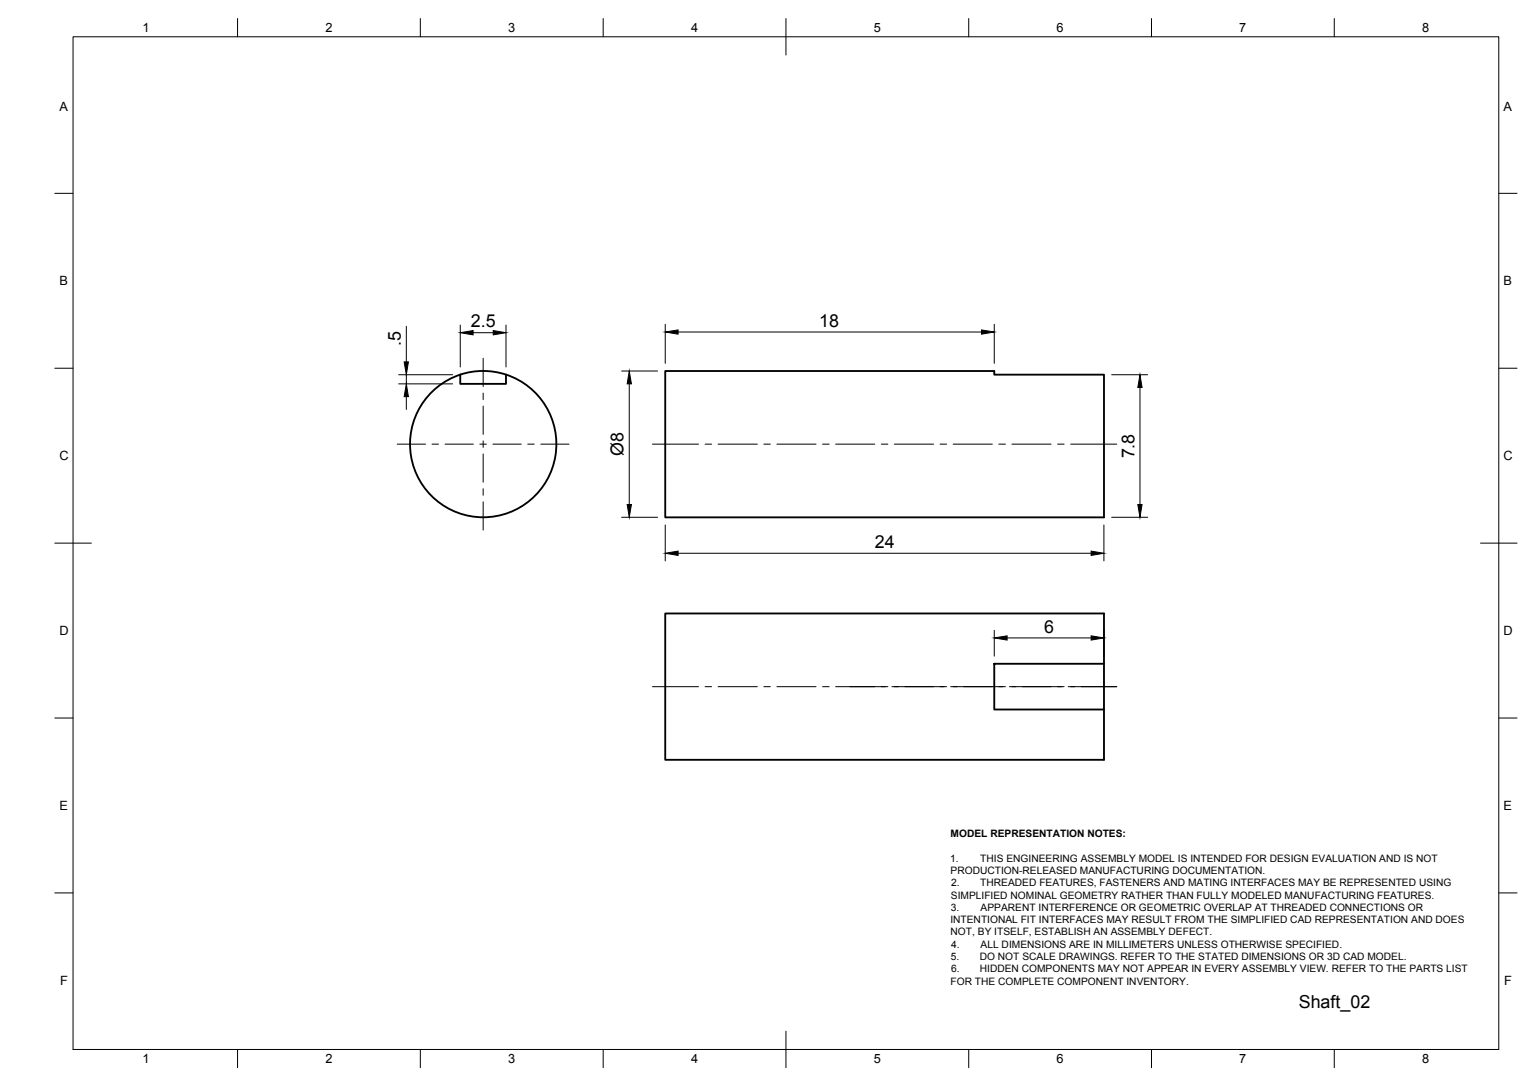
ISO-10303-21;
HEADER;
/* Generated by software containing ST-Developer
 * from STEP Tools, Inc. (www.steptools.com) 
 */

FILE_DESCRIPTION(
/* description */ (''),
/* implementation_level */ '2;1');

FILE_NAME(
/* name */ 'Shaft_02.step',
/* time_stamp */ '2026-10-05T22:24:12-07:00',
/* author */ (''),
/* organization */ (''),
/* preprocessor_version */ 'ST-DEVELOPER v20.2',
/* originating_system */ 'Autodesk Translation Framework v15.15.0.0',
/* authorisation */ '');

FILE_SCHEMA (('AUTOMOTIVE_DESIGN { 1 0 10303 214 3 1 1 }'));
ENDSEC;

DATA;
#10=MECHANICAL_DESIGN_GEOMETRIC_PRESENTATION_REPRESENTATION('',(#56),#2116);
#42=SHAPE_REPRESENTATION_RELATIONSHIP('SRR','None',#2148,#49);
#49=ADVANCED_BREP_SHAPE_REPRESENTATION('',(#63),#2112);
#56=STYLED_ITEM('',(#2192),#63);
#63=MANIFOLD_SOLID_BREP('Body1',#1150);
#107=PLANE('',#1310);
#108=PLANE('',#1311);
#109=PLANE('',#1312);
#110=PLANE('',#1313);
#111=PLANE('',#1315);
#112=PLANE('',#1320);
#172=FACE_OUTER_BOUND('',#247,.T.);
#173=FACE_OUTER_BOUND('',#248,.T.);
#174=FACE_OUTER_BOUND('',#249,.T.);
#175=FACE_OUTER_BOUND('',#250,.T.);
#176=FACE_OUTER_BOUND('',#251,.T.);
#177=FACE_OUTER_BOUND('',#252,.T.);
#178=FACE_OUTER_BOUND('',#253,.T.);
#247=EDGE_LOOP('',(#961,#962,#963,#964));
#248=EDGE_LOOP('',(#965,#966,#967,#968));
#249=EDGE_LOOP('',(#969,#970,#971,#972));
#250=EDGE_LOOP('',(#973,#974,#975,#976));
#251=EDGE_LOOP('',(#977,#978,#979,#980,#981));
#252=EDGE_LOOP('',(#982,#983,#984,#985,#986,#987,#988,#989));
#253=EDGE_LOOP('',(#990));
#335=LINE('',#1976,#440);
#336=LINE('',#1978,#441);
#337=LINE('',#1980,#442);
#338=LINE('',#1981,#443);
#339=LINE('',#1984,#444);
#340=LINE('',#1986,#445);
#341=LINE('',#1987,#446);
#342=LINE('',#1991,#447);
#343=LINE('',#1992,#448);
#344=LINE('',#1993,#449);
#345=LINE('',#2002,#450);
#440=VECTOR('',#1571,10.);
#441=VECTOR('',#1572,10.);
#442=VECTOR('',#1573,10.);
#443=VECTOR('',#1574,10.);
#444=VECTOR('',#1577,10.);
#445=VECTOR('',#1578,10.);
#446=VECTOR('',#1579,10.);
#447=VECTOR('',#1582,10.);
#448=VECTOR('',#1583,10.);
#449=VECTOR('',#1584,10.);
#450=VECTOR('',#1597,4.);
#518=CIRCLE('',#1314,4.);
#519=CIRCLE('',#1316,4.);
#520=CIRCLE('',#1317,4.);
#521=CIRCLE('',#1319,4.);
#589=VERTEX_POINT('',#1974);
#590=VERTEX_POINT('',#1975);
#591=VERTEX_POINT('',#1977);
#592=VERTEX_POINT('',#1979);
#593=VERTEX_POINT('',#1983);
#594=VERTEX_POINT('',#1985);
#595=VERTEX_POINT('',#1989);
#596=VERTEX_POINT('',#1990);
#597=VERTEX_POINT('',#1997);
#598=VERTEX_POINT('',#2001);
#719=EDGE_CURVE('',#589,#590,#335,.T.);
#720=EDGE_CURVE('',#591,#589,#336,.T.);
#721=EDGE_CURVE('',#592,#591,#337,.T.);
#722=EDGE_CURVE('',#590,#592,#338,.T.);
#723=EDGE_CURVE('',#592,#593,#339,.T.);
#724=EDGE_CURVE('',#594,#591,#340,.T.);
#725=EDGE_CURVE('',#593,#594,#341,.T.);
#726=EDGE_CURVE('',#595,#596,#342,.T.);
#727=EDGE_CURVE('',#593,#595,#343,.T.);
#728=EDGE_CURVE('',#596,#594,#344,.T.);
#729=EDGE_CURVE('',#596,#589,#518,.T.);
#730=EDGE_CURVE('',#595,#597,#519,.T.);
#731=EDGE_CURVE('',#597,#590,#520,.T.);
#732=EDGE_CURVE('',#597,#598,#345,.T.);
#733=EDGE_CURVE('',#598,#598,#521,.T.);
#961=ORIENTED_EDGE('',*,*,#719,.F.);
#962=ORIENTED_EDGE('',*,*,#720,.F.);
#963=ORIENTED_EDGE('',*,*,#721,.F.);
#964=ORIENTED_EDGE('',*,*,#722,.F.);
#965=ORIENTED_EDGE('',*,*,#723,.F.);
#966=ORIENTED_EDGE('',*,*,#721,.T.);
#967=ORIENTED_EDGE('',*,*,#724,.F.);
#968=ORIENTED_EDGE('',*,*,#725,.F.);
#969=ORIENTED_EDGE('',*,*,#726,.F.);
#970=ORIENTED_EDGE('',*,*,#727,.F.);
#971=ORIENTED_EDGE('',*,*,#725,.T.);
#972=ORIENTED_EDGE('',*,*,#728,.F.);
#973=ORIENTED_EDGE('',*,*,#729,.F.);
#974=ORIENTED_EDGE('',*,*,#728,.T.);
#975=ORIENTED_EDGE('',*,*,#724,.T.);
#976=ORIENTED_EDGE('',*,*,#720,.T.);
#977=ORIENTED_EDGE('',*,*,#722,.T.);
#978=ORIENTED_EDGE('',*,*,#723,.T.);
#979=ORIENTED_EDGE('',*,*,#727,.T.);
#980=ORIENTED_EDGE('',*,*,#730,.T.);
#981=ORIENTED_EDGE('',*,*,#731,.T.);
#982=ORIENTED_EDGE('',*,*,#730,.F.);
#983=ORIENTED_EDGE('',*,*,#726,.T.);
#984=ORIENTED_EDGE('',*,*,#729,.T.);
#985=ORIENTED_EDGE('',*,*,#719,.T.);
#986=ORIENTED_EDGE('',*,*,#731,.F.);
#987=ORIENTED_EDGE('',*,*,#732,.T.);
#988=ORIENTED_EDGE('',*,*,#733,.T.);
#989=ORIENTED_EDGE('',*,*,#732,.F.);
#990=ORIENTED_EDGE('',*,*,#733,.F.);
#1078=CYLINDRICAL_SURFACE('',#1318,4.);
#1121=ADVANCED_FACE('',(#172),#107,.T.);
#1122=ADVANCED_FACE('',(#173),#108,.T.);
#1123=ADVANCED_FACE('',(#174),#109,.T.);
#1124=ADVANCED_FACE('',(#175),#110,.T.);
#1125=ADVANCED_FACE('',(#176),#111,.T.);
#1126=ADVANCED_FACE('',(#177),#1078,.T.);
#1127=ADVANCED_FACE('',(#178),#112,.F.);
#1150=CLOSED_SHELL('',(#1121,#1122,#1123,#1124,#1125,#1126,#1127));
#1309=AXIS2_PLACEMENT_3D('',#1972,#1567,#1568);
#1310=AXIS2_PLACEMENT_3D('',#1973,#1569,#1570);
#1311=AXIS2_PLACEMENT_3D('',#1982,#1575,#1576);
#1312=AXIS2_PLACEMENT_3D('',#1988,#1580,#1581);
#1313=AXIS2_PLACEMENT_3D('',#1994,#1585,#1586);
#1314=AXIS2_PLACEMENT_3D('',#1995,#1587,#1588);
#1315=AXIS2_PLACEMENT_3D('',#1996,#1589,#1590);
#1316=AXIS2_PLACEMENT_3D('',#1998,#1591,#1592);
#1317=AXIS2_PLACEMENT_3D('',#1999,#1593,#1594);
#1318=AXIS2_PLACEMENT_3D('',#2000,#1595,#1596);
#1319=AXIS2_PLACEMENT_3D('',#2003,#1598,#1599);
#1320=AXIS2_PLACEMENT_3D('',#2004,#1600,#1601);
#1567=DIRECTION('axis',(0.,0.,1.));
#1568=DIRECTION('refdir',(1.,0.,0.));
#1569=DIRECTION('center_axis',(-1.,0.,0.));
#1570=DIRECTION('ref_axis',(0.,0.,1.));
#1571=DIRECTION('',(0.,-1.,0.));
#1572=DIRECTION('',(0.,0.,1.));
#1573=DIRECTION('',(0.,1.,0.));
#1574=DIRECTION('',(0.,0.,-1.));
#1575=DIRECTION('center_axis',(0.,0.,1.));
#1576=DIRECTION('ref_axis',(1.,0.,0.));
#1577=DIRECTION('',(-1.,0.,0.));
#1578=DIRECTION('',(1.,0.,0.));
#1579=DIRECTION('',(0.,1.,0.));
#1580=DIRECTION('center_axis',(1.,0.,0.));
#1581=DIRECTION('ref_axis',(0.,0.,-1.));
#1582=DIRECTION('',(0.,1.,0.));
#1583=DIRECTION('',(0.,0.,1.));
#1584=DIRECTION('',(0.,0.,-1.));
#1585=DIRECTION('center_axis',(0.,-1.,0.));
#1586=DIRECTION('ref_axis',(0.,0.,-1.));
#1587=DIRECTION('center_axis',(0.,1.,0.));
#1588=DIRECTION('ref_axis',(1.,0.,0.));
#1589=DIRECTION('center_axis',(0.,-1.,0.));
#1590=DIRECTION('ref_axis',(1.,0.,0.));
#1591=DIRECTION('center_axis',(0.,-1.,0.));
#1592=DIRECTION('ref_axis',(1.,0.,0.));
#1593=DIRECTION('center_axis',(0.,-1.,0.));
#1594=DIRECTION('ref_axis',(1.,0.,0.));
#1595=DIRECTION('center_axis',(0.,-1.,0.));
#1596=DIRECTION('ref_axis',(1.,0.,0.));
#1597=DIRECTION('',(0.,1.,0.));
#1598=DIRECTION('center_axis',(0.,-1.,0.));
#1599=DIRECTION('ref_axis',(1.,0.,0.));
#1600=DIRECTION('center_axis',(0.,-1.,0.));
#1601=DIRECTION('ref_axis',(1.,0.,0.));
#1972=CARTESIAN_POINT('',(0.,0.,0.));
#1973=CARTESIAN_POINT('Origin',(3.25,10.,5.29967103839267));
#1974=CARTESIAN_POINT('',(3.25,16.,5.79967103839267));
#1975=CARTESIAN_POINT('',(3.25,10.,5.79967103839267));
#1976=CARTESIAN_POINT('',(3.25,10.,5.79967103839267));
#1977=CARTESIAN_POINT('',(3.25,16.,5.29967103839267));
#1978=CARTESIAN_POINT('',(3.25,16.,8.32461990770089));
#1979=CARTESIAN_POINT('',(3.25,10.,5.29967103839267));
#1980=CARTESIAN_POINT('',(3.25,10.,5.29967103839267));
#1981=CARTESIAN_POINT('',(3.25,10.,3.64983551919633));
#1982=CARTESIAN_POINT('Origin',(0.75,10.,5.29967103839267));
#1983=CARTESIAN_POINT('',(0.75,10.,5.29967103839267));
#1984=CARTESIAN_POINT('',(1.375,10.,5.29967103839267));
#1985=CARTESIAN_POINT('',(0.75,16.,5.29967103839267));
#1986=CARTESIAN_POINT('',(0.75,16.,5.29967103839267));
#1987=CARTESIAN_POINT('',(0.75,10.,5.29967103839267));
#1988=CARTESIAN_POINT('Origin',(0.75,10.,6.84122918275927));
#1989=CARTESIAN_POINT('',(0.75,10.,5.79967103839267));
#1990=CARTESIAN_POINT('',(0.75,16.,5.79967103839267));
#1991=CARTESIAN_POINT('',(0.75,10.,5.79967103839267));
#1992=CARTESIAN_POINT('',(0.75,10.,4.42061459137964));
#1993=CARTESIAN_POINT('',(0.75,16.,5.79967103839267));
#1994=CARTESIAN_POINT('Origin',(2.,16.,6.07045011057597));
#1995=CARTESIAN_POINT('Origin',(2.,16.,2.));
#1996=CARTESIAN_POINT('Origin',(2.,10.,2.));
#1997=CARTESIAN_POINT('',(-2.,10.,2.));
#1998=CARTESIAN_POINT('Origin',(2.,10.,2.));
#1999=CARTESIAN_POINT('Origin',(2.,10.,2.));
#2000=CARTESIAN_POINT('Origin',(2.,10.,2.));
#2001=CARTESIAN_POINT('',(-2.,34.,2.));
#2002=CARTESIAN_POINT('',(-2.,10.,2.));
#2003=CARTESIAN_POINT('Origin',(2.,34.,2.));
#2004=CARTESIAN_POINT('Origin',(2.,34.,2.));
#2103=UNCERTAINTY_MEASURE_WITH_UNIT(LENGTH_MEASURE(0.01),#2117,
'DISTANCE_ACCURACY_VALUE',
'Maximum model space distance between geometric entities at asserted c
onnectivities');
#2107=UNCERTAINTY_MEASURE_WITH_UNIT(LENGTH_MEASURE(0.01),#2117,
'DISTANCE_ACCURACY_VALUE',
'Maximum model space distance between geometric entities at asserted c
onnectivities');
#2112=(
GEOMETRIC_REPRESENTATION_CONTEXT(3)
GLOBAL_UNCERTAINTY_ASSIGNED_CONTEXT((#2103))
GLOBAL_UNIT_ASSIGNED_CONTEXT((#2117,#2119,#2120))
REPRESENTATION_CONTEXT('','3D')
);
#2116=(
GEOMETRIC_REPRESENTATION_CONTEXT(3)
GLOBAL_UNCERTAINTY_ASSIGNED_CONTEXT((#2107))
GLOBAL_UNIT_ASSIGNED_CONTEXT((#2117,#2119,#2120))
REPRESENTATION_CONTEXT('','3D')
);
#2117=(
LENGTH_UNIT()
NAMED_UNIT(*)
SI_UNIT(.MILLI.,.METRE.)
);
#2119=(
NAMED_UNIT(*)
PLANE_ANGLE_UNIT()
SI_UNIT($,.RADIAN.)
);
#2120=(
NAMED_UNIT(*)
SI_UNIT($,.STERADIAN.)
SOLID_ANGLE_UNIT()
);
#2125=SHAPE_DEFINITION_REPRESENTATION(#2133,#2148);
#2133=PRODUCT_DEFINITION_SHAPE('',$,#2157);
#2148=SHAPE_REPRESENTATION('',(#1309),#2112);
#2152=PRODUCT_DEFINITION_CONTEXT('part definition',#2178,'design');
#2157=PRODUCT_DEFINITION('Shaft_02','Shaft_02',#2165,#2152);
#2165=PRODUCT_DEFINITION_FORMATION('',$,#2184);
#2178=APPLICATION_CONTEXT(
'Core Data for Automotive Mechanical Design Process');
#2179=PRODUCT_CONTEXT('part definition',#2178,'mechanical');
#2184=PRODUCT('Shaft_02','Shaft_02',$,(#2179));
#2192=PRESENTATION_STYLE_ASSIGNMENT((#2197));
#2197=SURFACE_STYLE_USAGE(.BOTH.,#2202);
#2202=SURFACE_SIDE_STYLE('',(#2207));
#2207=SURFACE_STYLE_FILL_AREA(#2212);
#2212=FILL_AREA_STYLE('Opaque(235,235,235)',(#2217));
#2217=FILL_AREA_STYLE_COLOUR('Opaque(235,235,235)',#2222);
#2222=COLOUR_RGB('Opaque(235,235,235)', 0.40784314, 0.44705882, 0.49803922);
ENDSEC;
END-ISO-10303-21;
